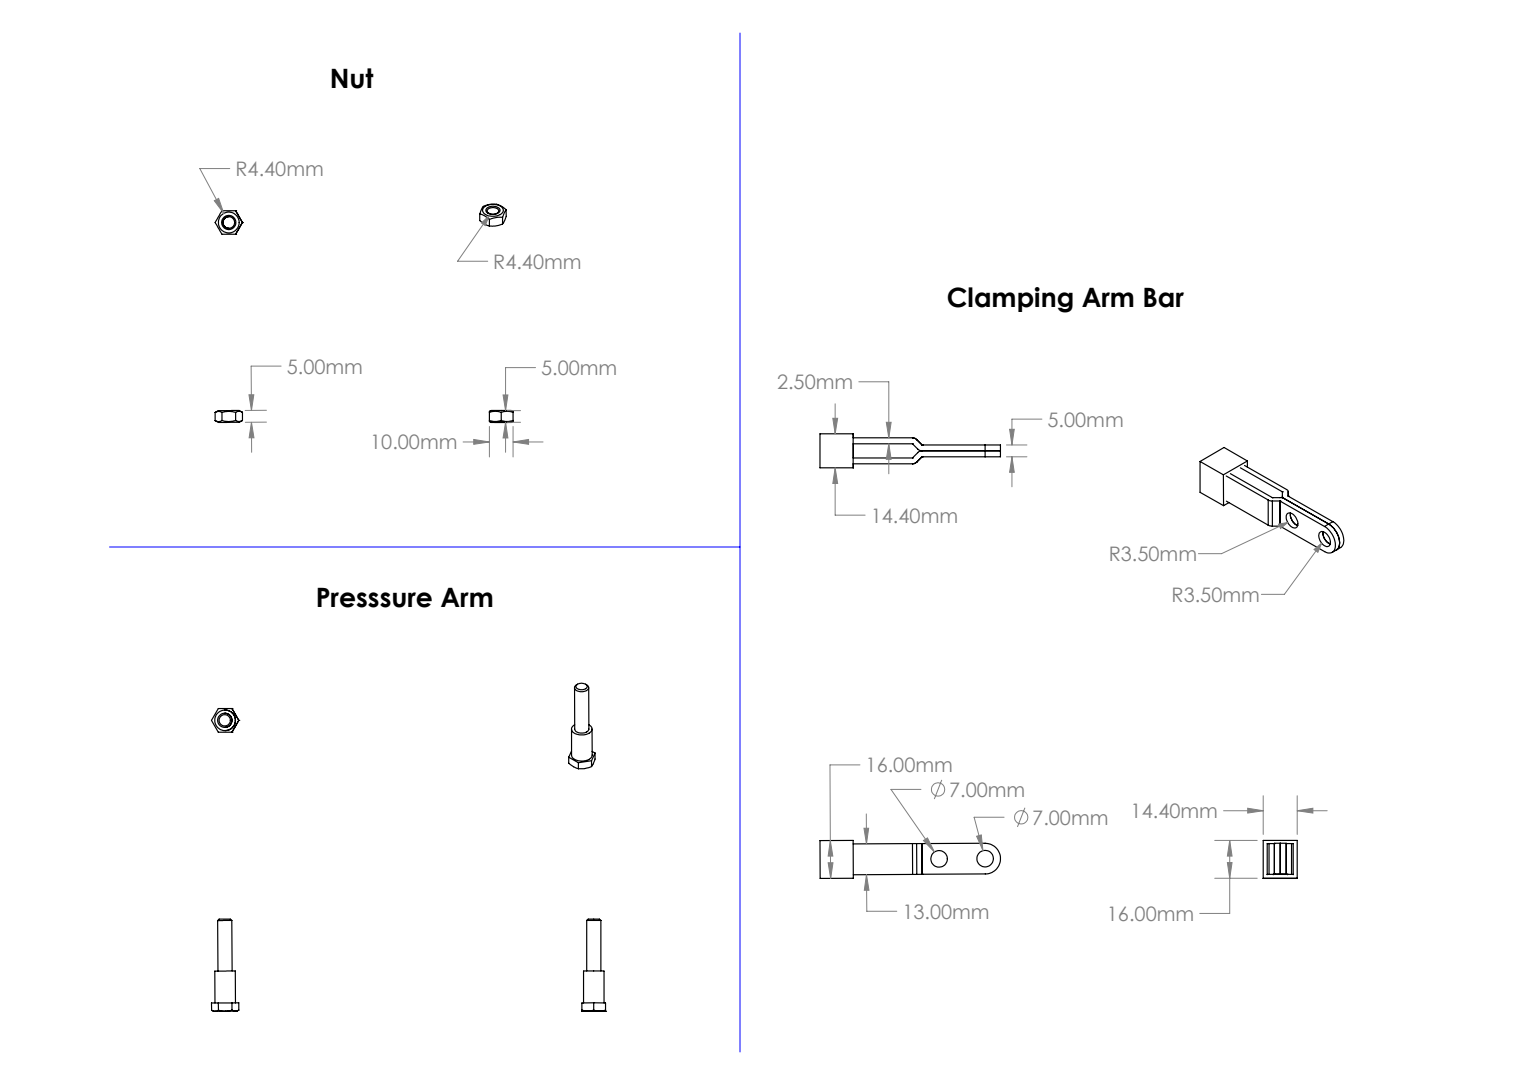
ISO-10303-21;
HEADER;
FILE_DESCRIPTION (('STEP AP203'),
    '1' );
FILE_NAME ('Nut.step',
    '2026-10-31T14:11:27',
    ( '' ),
    ( '' ),
    'SwSTEP 2.0',
    'SolidWorks 2024',
    '' );
FILE_SCHEMA (( 'AUTOMOTIVE_DESIGN' ));
ENDSEC;

DATA;
#48=ORIENTED_EDGE ( 'NONE', *, *, #17410, .F. ) ;
#83=EDGE_CURVE ( 'NONE', #7095, #13655, #23162, .T. ) ;
#118=EDGE_CURVE ( 'NONE', #1889, #6893, #1553, .T. ) ;
#162=CARTESIAN_POINT ( 'NONE',  ( -62.91331795724000386, 7.826945432762889787, -2.729132938682638176 ) ) ;
#166=DIRECTION ( 'NONE',  ( -0.005235963827117092427, 0.9999862922474493931, 2.636227439667000721E-16 ) ) ;
#193=ADVANCED_FACE ( 'NONE', ( #7501 ), #14386, .T. ) ;
#202=VECTOR ( 'NONE', #1831, 1000.000000000000114 ) ;
#242=ORIENTED_EDGE ( 'NONE', *, *, #2441, .T. ) ;
#415=DIRECTION ( 'NONE',  ( 1.000000000000000000, 0.000000000000000000, 0.000000000000000000 ) ) ;
#502=CONICAL_SURFACE ( 'NONE', #13794, 5.086751345948125724, 1.047197551196598297 ) ;
#564=ORIENTED_EDGE ( 'NONE', *, *, #13143, .F. ) ;
#585=ORIENTED_EDGE ( 'NONE', *, *, #14857, .F. ) ;
#607=DIRECTION ( 'NONE',  ( 0.002617981913558544045, -0.4999931461237241970, 0.8660254037844389297 ) ) ;
#658=ORIENTED_EDGE ( 'NONE', *, *, #17806, .F. ) ;
#748=FACE_OUTER_BOUND ( 'NONE', #10952, .T. ) ;
#759=FACE_OUTER_BOUND ( 'NONE', #8921, .T. ) ;
#769=CIRCLE ( 'NONE', #12189, 2.999765877365279998 ) ;
#838=ORIENTED_EDGE ( 'NONE', *, *, #7929, .T. ) ;
#909=( BOUNDED_CURVE ( )  B_SPLINE_CURVE ( 2, ( #15250, #2658, #18475 ),
 .UNSPECIFIED., .F., .F. ) 
 B_SPLINE_CURVE_WITH_KNOTS ( ( 3, 3 ),
 ( 0.000000000000000000, 0.5842180690389598974 ),
 .UNSPECIFIED. ) 
 CURVE ( )  GEOMETRIC_REPRESENTATION_ITEM ( )  RATIONAL_B_SPLINE_CURVE ( ( 1.000000000000000000, 1.154700538379259900, 1.000000000000000000 ) ) 
 REPRESENTATION_ITEM ( '' )  );
#924=APPLICATION_CONTEXT ( 'configuration controlled 3d designs of mechanical parts and assemblies' ) ;
#950=EDGE_CURVE ( 'NONE', #15424, #21777, #11621, .T. ) ;
#1004=DIRECTION ( 'NONE',  ( 0.000000000000000000, 0.000000000000000000, -1.000000000000000000 ) ) ;
#1008=VERTEX_POINT ( 'NONE', #8728 ) ;
#1066=ORIENTED_EDGE ( 'NONE', *, *, #2450, .T. ) ;
#1074=MECHANICAL_CONTEXT ( 'NONE', #3800, 'mechanical' ) ;
#1122=VECTOR ( 'NONE', #13490, 1000.000000000000114 ) ;
#1158=ORIENTED_EDGE ( 'NONE', *, *, #13143, .T. ) ;
#1192=ORIENTED_EDGE ( 'NONE', *, *, #14770, .T. ) ;
#1220=CARTESIAN_POINT ( 'NONE',  ( -62.91249983789198552, 7.670697574599230073, 2.108981951733699973E-15 ) ) ;
#1228=DIRECTION ( 'NONE',  ( 0.005235963827117092427, -0.9999862922474493931, -2.636227439667000721E-16 ) ) ;
#1258=( BOUNDED_CURVE ( )  B_SPLINE_CURVE ( 2, ( #13455, #15223, #2276 ),
 .UNSPECIFIED., .F., .F. ) 
 B_SPLINE_CURVE_WITH_KNOTS ( ( 3, 3 ),
 ( 0.000000000000000000, 0.5842180690389568998 ),
 .UNSPECIFIED. ) 
 CURVE ( )  GEOMETRIC_REPRESENTATION_ITEM ( )  RATIONAL_B_SPLINE_CURVE ( ( 1.000000000000000000, 1.154700538379249908, 1.000000000000000000 ) ) 
 REPRESENTATION_ITEM ( '' )  );
#1289=EDGE_LOOP ( 'NONE', ( #838, #3310, #5505, #18636 ) ) ;
#1334=CARTESIAN_POINT ( 'NONE',  ( -65.82539143210260590, 12.65551411021120032, 5.000000000000000000 ) ) ;
#1422=DIRECTION ( 'NONE',  ( 0.005235963827117092427, -0.9999862922474493931, -2.636227439667000721E-16 ) ) ;
#1439=CARTESIAN_POINT ( 'NONE',  ( -62.99678855639989905, 23.76850991288289805, -2.458499999999993690 ) ) ;
#1553=LINE ( 'NONE', #17616, #5745 ) ;
#1701=EDGE_LOOP ( 'NONE', ( #19939, #14934, #11313, #2927 ) ) ;
#1743=CARTESIAN_POINT ( 'NONE',  ( -62.93704341833160498, 12.35813331950920002, 2.458500000000117147 ) ) ;
#1749=DIRECTION ( 'NONE',  ( 0.9999862922474493931, 0.005235963827117055998, -1.750845403988397166E-31 ) ) ;
#1818=ORIENTED_EDGE ( 'NONE', *, *, #13921, .T. ) ;
#1831=DIRECTION ( 'NONE',  ( 0.002617981913558435191, -0.4999931461237237529, -0.8660254037844391517 ) ) ;
#1866=DIRECTION ( 'NONE',  ( 0.000000000000000000, 0.000000000000000000, -1.000000000000000000 ) ) ;
#1873=CARTESIAN_POINT ( 'NONE',  ( -57.16525610687759951, 12.70085888708699962, 5.715859474400029324E-15 ) ) ;
#1889=VERTEX_POINT ( 'NONE', #4406 ) ;
#1933=MANIFOLD_SOLID_BREP ( 'Imported1', #14367 ) ;
#2181=DIRECTION ( 'NONE',  ( -2.065223582182029992E-34, 2.636263576915770120E-16, -1.000000000000000000 ) ) ;
#2264=( GEOMETRIC_REPRESENTATION_CONTEXT ( 3 ) GLOBAL_UNCERTAINTY_ASSIGNED_CONTEXT ( ( #7928 ) ) GLOBAL_UNIT_ASSIGNED_CONTEXT ( ( #4646, #11789, #6547 ) ) REPRESENTATION_CONTEXT ( 'NONE', 'WORKASPACE' ) );
#2276=CARTESIAN_POINT ( 'NONE',  ( -60.04781580374580585, 11.89276268270289982, -5.000000000000000000 ) ) ;
#2301=DIRECTION ( 'NONE',  ( 0.005235963827117091560, -0.9999862922474493931, -2.636227439666999735E-16 ) ) ;
#2397=CIRCLE ( 'NONE', #19868, 4.399999999999997691 ) ;
#2419=ORIENTED_EDGE ( 'NONE', *, *, #15064, .T. ) ;
#2441=EDGE_CURVE ( 'NONE', #13655, #6050, #20011, .T. ) ;
#2450=EDGE_CURVE ( 'NONE', #13217, #14219, #21981, .T. ) ;
#2491=CARTESIAN_POINT ( 'NONE',  ( -57.16525610687759951, 12.70085888708699962, 5.715859474400029324E-15 ) ) ;
#2514=CARTESIAN_POINT ( 'NONE',  ( -65.82539143210260590, 12.65551411021120032, 5.000000000000000000 ) ) ;
#2569=CARTESIAN_POINT ( 'NONE',  ( 0.000000000000000000, 0.000000000000000000, 0.000000000000000000 ) ) ;
#2587=( BOUNDED_CURVE ( )  B_SPLINE_CURVE ( 2, ( #19385, #13684, #8344 ),
 .UNSPECIFIED., .F., .T. ) 
 B_SPLINE_CURVE_WITH_KNOTS ( ( 3, 3 ),
 ( 0.000000000000000000, 0.5842180690389588982 ),
 .UNSPECIFIED. ) 
 CURVE ( )  GEOMETRIC_REPRESENTATION_ITEM ( )  RATIONAL_B_SPLINE_CURVE ( ( 1.000000000000000000, 1.154700538379249908, 1.000000000000000000 ) ) 
 REPRESENTATION_ITEM ( '' )  );
#2605=EDGE_CURVE ( 'NONE', #22018, #17928, #909, .T. ) ;
#2653=AXIS2_PLACEMENT_3D ( 'NONE', #22839, #8363, #3007 ) ;
#2658=CARTESIAN_POINT ( 'NONE',  ( -67.24235627552212691, 7.607684554713951997, -2.500000000000000000 ) ) ;
#2677=CARTESIAN_POINT ( 'NONE',  ( -67.33861934291638818, 12.64759079499718375, 3.945395128240059864E-15 ) ) ;
#2734=ORIENTED_EDGE ( 'NONE', *, *, #4247, .F. ) ;
#2762=CARTESIAN_POINT ( 'NONE',  ( -62.99678855639989905, 23.76850991288289805, 2.458500000000006569 ) ) ;
#2799=ORIENTED_EDGE ( 'NONE', *, *, #10035, .T. ) ;
#2808=AXIS2_PLACEMENT_3D ( 'NONE', #14494, #21733, #5472 ) ;
#2809=ADVANCED_FACE ( 'NONE', ( #6343 ), #10163, .T. ) ;
#2822=EDGE_CURVE ( 'NONE', #1008, #6050, #7463, .T. ) ;
#2848=CARTESIAN_POINT ( 'NONE',  ( -60.04781580374580585, 11.89276268270289982, 5.000000000000000000 ) ) ;
#2856=ADVANCED_BREP_SHAPE_REPRESENTATION ( '', ( #1933, #12739 ), #2264 ) ;
#2927=ORIENTED_EDGE ( 'NONE', *, *, #18076, .T. ) ;
#2955=CARTESIAN_POINT ( 'NONE',  ( -60.04781580374580585, 11.89276268270289982, 5.000000000000000000 ) ) ;
#2961=DIRECTION ( 'NONE',  ( -0.005235963827117092427, 0.9999862922474493931, 2.636227439667000721E-16 ) ) ;
#3007=DIRECTION ( 'NONE',  ( 0.9999862922474493931, 0.005235963827117055998, -1.750845403988397166E-31 ) ) ;
#3099=ORIENTED_EDGE ( 'NONE', *, *, #10881, .F. ) ;
#3193=EDGE_CURVE ( 'NONE', #17928, #13217, #16240, .T. ) ;
#3195=CARTESIAN_POINT ( 'NONE',  ( -68.69007546624879978, 8.433449002107520798, 2.873144230283079984E-15 ) ) ;
#3310=ORIENTED_EDGE ( 'NONE', *, *, #950, .T. ) ;
#3325=FACE_OUTER_BOUND ( 'NONE', #4037, .T. ) ;
#3450=CARTESIAN_POINT ( 'NONE',  ( -62.99678855639989905, 23.76850991288289805, 6.352789585277969841E-15 ) ) ;
#3602=CARTESIAN_POINT ( 'NONE',  ( -67.26895854462254931, 12.68829727884599201, -2.499999999999999556 ) ) ;
#3687=AXIS2_PLACEMENT_3D ( 'NONE', #13492, #20727, #5393 ) ;
#3754=DIRECTION ( 'NONE',  ( 0.9999862922474491711, 0.005235963827117207786, -1.514467536079854800E-31 ) ) ;
#3762=ORIENTED_EDGE ( 'NONE', *, *, #4612, .F. ) ;
#3800=APPLICATION_CONTEXT ( 'configuration controlled 3d designs of mechanical parts and assemblies' ) ;
#3801=DIRECTION ( 'NONE',  ( 0.005235963827117092427, -0.9999862922474493931, -2.636227439667000721E-16 ) ) ;
#3816=ADVANCED_FACE ( 'NONE', ( #5637 ), #12564, .F. ) ;
#3882=AXIS2_PLACEMENT_3D ( 'NONE', #15257, #11723, #9577 ) ;
#4033=DIRECTION ( 'NONE',  ( 0.005235963827117092427, -0.9999862922474493931, -2.636227439667000721E-16 ) ) ;
#4037=EDGE_LOOP ( 'NONE', ( #2734, #6715, #5931, #12250 ) ) ;
#4108=CARTESIAN_POINT ( 'NONE',  ( -65.80336369117380002, 8.448563927732790191, -5.000000000000000000 ) ) ;
#4131=FACE_OUTER_BOUND ( 'NONE', #11927, .T. ) ;
#4152=CARTESIAN_POINT ( 'NONE',  ( -58.58222095029707077, 7.653029331589754847, 2.499999999999999556 ) ) ;
#4184=CARTESIAN_POINT ( 'NONE',  ( -68.71210320717760567, 12.64039918458589895, 4.433884350144319916E-15 ) ) ;
#4247=EDGE_CURVE ( 'NONE', #15424, #7095, #16030, .T. ) ;
#4308=ORIENTED_EDGE ( 'NONE', *, *, #10796, .T. ) ;
#4336=FACE_OUTER_BOUND ( 'NONE', #12032, .T. ) ;
#4406=CARTESIAN_POINT ( 'NONE',  ( -58.51256015200321059, 7.693735815438545345, 2.108981951733699184E-15 ) ) ;
#4413=LINE ( 'NONE', #2514, #14045 ) ;
#4482=EDGE_CURVE ( 'NONE', #15538, #1008, #9896, .T. ) ;
#4520=CARTESIAN_POINT ( 'NONE',  ( -60.04781580374580585, 11.89276268270289982, -5.000000000000000000 ) ) ;
#4546=AXIS2_PLACEMENT_3D ( 'NONE', #13889, #2961, #6776 ) ;
#4568=ADVANCED_FACE ( 'NONE', ( #22220 ), #5965, .T. ) ;
#4593=( BOUNDED_CURVE ( )  B_SPLINE_CURVE ( 2, ( #9269, #9752, #20191 ),
 .UNSPECIFIED., .F., .F. ) 
 B_SPLINE_CURVE_WITH_KNOTS ( ( 3, 3 ),
 ( 0.000000000000000000, 0.5842180690389568998 ),
 .UNSPECIFIED. ) 
 CURVE ( )  GEOMETRIC_REPRESENTATION_ITEM ( )  RATIONAL_B_SPLINE_CURVE ( ( 1.000000000000000000, 1.154700538379249908, 1.000000000000000000 ) ) 
 REPRESENTATION_ITEM ( '' )  );
#4612=EDGE_CURVE ( 'NONE', #15424, #15538, #15813, .T. ) ;
#4618=VECTOR ( 'NONE', #15931, 1000.000000000000000 ) ;
#4630=DIRECTION ( 'NONE',  ( -0.002617981913558544045, 0.4999931461237241970, -0.8660254037844389297 ) ) ;
#4646=( LENGTH_UNIT ( ) NAMED_UNIT ( * ) SI_UNIT ( .MILLI., .METRE. ) );
#4714=ORIENTED_EDGE ( 'NONE', *, *, #3193, .F. ) ;
#4771=LINE ( 'NONE', #16801, #18748 ) ;
#4897=CARTESIAN_POINT ( 'NONE',  ( -65.82123935389580538, 11.86253283145240012, 5.000000000000000000 ) ) ;
#5071=CARTESIAN_POINT ( 'NONE',  ( -62.91413607658799378, 7.983193290926558383, 2.191364059223300011E-15 ) ) ;
#5115=CARTESIAN_POINT ( 'NONE',  ( -62.99678855639989905, 23.76850991288289805, 6.352789585277969841E-15 ) ) ;
#5160=EDGE_CURVE ( 'NONE', #21777, #22844, #7220, .T. ) ;
#5174=DIRECTION ( 'NONE',  ( 0.000000000000000000, 0.000000000000000000, 1.000000000000000000 ) ) ;
#5204=CARTESIAN_POINT ( 'NONE',  ( -67.24235627552209849, 7.607684554713948444, 2.499999999999999556 ) ) ;
#5240=EDGE_CURVE ( 'NONE', #7095, #22844, #15320, .T. ) ;
#5281=CARTESIAN_POINT ( 'NONE',  ( -60.02994014102380049, 8.478793778983318319, -5.000000000000000000 ) ) ;
#5326=CARTESIAN_POINT ( 'NONE',  ( -57.14322836594880073, 8.493908704608589488, 2.318032717970499742E-15 ) ) ;
#5393=DIRECTION ( 'NONE',  ( 6.009176021521548497E-19, -0.9999588795606765279, 0.009068582455730085992 ) ) ;
#5433=CARTESIAN_POINT ( 'NONE',  ( -62.93660361792420588, 12.27413839645710070, 3.322570288448809768E-15 ) ) ;
#5438=AXIS2_PLACEMENT_3D ( 'NONE', #9077, #23323, #11120 ) ;
#5472=DIRECTION ( 'NONE',  ( 0.000000000000000000, 0.000000000000000000, 1.000000000000000000 ) ) ;
#5505=ORIENTED_EDGE ( 'NONE', *, *, #5160, .T. ) ;
#5618=ORIENTED_EDGE ( 'NONE', *, *, #21166, .F. ) ;
#5637=FACE_OUTER_BOUND ( 'NONE', #1701, .T. ) ;
#5745=VECTOR ( 'NONE', #8823, 1000.000000000000114 ) ;
#5757=CARTESIAN_POINT ( 'NONE',  ( -62.93786153767959490, 12.51438117767279934, 3.385904617822409831E-15 ) ) ;
#5783=FACE_OUTER_BOUND ( 'NONE', #17641, .T. ) ;
#5803=AXIS2_PLACEMENT_3D ( 'NONE', #9495, #19949, #14953 ) ;
#5818=AXIS2_PLACEMENT_3D ( 'NONE', #5115, #23377, #14247 ) ;
#5931=ORIENTED_EDGE ( 'NONE', *, *, #10263, .F. ) ;
#5965=PLANE ( 'NONE',  #15646 ) ;
#5993=FACE_BOUND ( 'NONE', #23430, .T. ) ;
#6034=CARTESIAN_POINT ( 'NONE',  ( -62.93704341833160498, 12.35813331950920002, -2.458500000000113150 ) ) ;
#6050=VERTEX_POINT ( 'NONE', #11465 ) ;
#6159=AXIS2_PLACEMENT_3D ( 'NONE', #11289, #10611, #18518 ) ;
#6199=EDGE_CURVE ( 'NONE', #11763, #11453, #2587, .T. ) ;
#6237=CARTESIAN_POINT ( 'NONE',  ( -60.02994014102380049, 8.478793778983318319, -5.000000000000000000 ) ) ;
#6239=FACE_OUTER_BOUND ( 'NONE', #9069, .T. ) ;
#6250=PLANE ( 'NONE',  #3687 ) ;
#6252=EDGE_CURVE ( 'NONE', #11453, #23172, #19441, .T. ) ;
#6318=CARTESIAN_POINT ( 'NONE',  ( -62.91331795724000386, 7.826945432762889787, 2.729132938682642617 ) ) ;
#6337=FACE_OUTER_BOUND ( 'NONE', #9256, .T. ) ;
#6343=FACE_OUTER_BOUND ( 'NONE', #13109, .T. ) ;
#6400=ORIENTED_EDGE ( 'NONE', *, *, #21166, .T. ) ;
#6414=CARTESIAN_POINT ( 'NONE',  ( -62.91331795724000386, 7.826945432762889787, 2.150173005478499992E-15 ) ) ;
#6491=EDGE_LOOP ( 'NONE', ( #9619, #22336, #18153, #15288 ) ) ;
#6547=( NAMED_UNIT ( * ) SI_UNIT ( $, .STERADIAN. ) SOLID_ANGLE_UNIT ( ) );
#6715=ORIENTED_EDGE ( 'NONE', *, *, #4612, .T. ) ;
#6776=DIRECTION ( 'NONE',  ( 0.000000000000000000, 0.000000000000000000, -1.000000000000000000 ) ) ;
#6793=ADVANCED_FACE ( 'NONE', ( #11913 ), #21721, .F. ) ;
#6797=CYLINDRICAL_SURFACE ( 'NONE', #21711, 2.458500000000000352 ) ;
#6893=VERTEX_POINT ( 'NONE', #5326 ) ;
#6975=PLANE ( 'NONE',  #5438 ) ;
#7032=FACE_OUTER_BOUND ( 'NONE', #11934, .T. ) ;
#7034=CARTESIAN_POINT ( 'NONE',  ( -65.82123935389580538, 11.86253283145240012, 5.000000000000000000 ) ) ;
#7095=VERTEX_POINT ( 'NONE', #6034 ) ;
#7220=CIRCLE ( 'NONE', #4546, 2.999765877365279998 ) ;
#7238=ORIENTED_EDGE ( 'NONE', *, *, #6199, .T. ) ;
#7257=AXIS2_PLACEMENT_3D ( 'NONE', #9569, #22596, #15367 ) ;
#7338=CIRCLE ( 'NONE', #5803, 2.458500000000000352 ) ;
#7358=DIRECTION ( 'NONE',  ( -0.005235963827117092427, 0.9999862922474493931, 2.636227439667000721E-16 ) ) ;
#7375=CIRCLE ( 'NONE', #2808, 2.458500000000000352 ) ;
#7377=ADVANCED_FACE ( 'NONE', ( #21653 ), #6975, .T. ) ;
#7463=CIRCLE ( 'NONE', #10513, 2.999765877365279998 ) ;
#7501=FACE_OUTER_BOUND ( 'NONE', #13056, .T. ) ;
#7530=ORIENTED_EDGE ( 'NONE', *, *, #14770, .F. ) ;
#7547=CIRCLE ( 'NONE', #16254, 4.399999999999997691 ) ;
#7614=PRODUCT_DEFINITION_FORMATION_WITH_SPECIFIED_SOURCE ( 'ANY', '', #21422, .NOT_KNOWN. ) ;
#7711=ADVANCED_FACE ( 'NONE', ( #3325 ), #16031, .F. ) ;
#7842=ORIENTED_EDGE ( 'NONE', *, *, #16626, .T. ) ;
#7879=DIRECTION ( 'NONE',  ( -0.005235963827117002221, 0.9999862922474493931, 2.636227439667000721E-16 ) ) ;
#7928=UNCERTAINTY_MEASURE_WITH_UNIT (LENGTH_MEASURE( 1.000000000000000082E-05 ), #4646, 'distance_accuracy_value', 'NONE');
#7929=EDGE_CURVE ( 'NONE', #7095, #15424, #7338, .T. ) ;
#8023=PLANE ( 'NONE',  #3882 ) ;
#8278=CARTESIAN_POINT ( 'NONE',  ( -62.91413607658799378, 7.983193290926554830, -2.458499999999998131 ) ) ;
#8326=ORIENTED_EDGE ( 'NONE', *, *, #17806, .T. ) ;
#8344=CARTESIAN_POINT ( 'NONE',  ( -65.82123935389580538, 11.86253283145240012, 5.000000000000000000 ) ) ;
#8363=DIRECTION ( 'NONE',  ( 0.005235963827117002221, -0.9999862922474493931, -2.636227439667000721E-16 ) ) ;
#8394=AXIS2_PLACEMENT_3D ( 'NONE', #5071, #10437, #5174 ) ;
#8521=ADVANCED_FACE ( 'NONE', ( #5783 ), #502, .T. ) ;
#8551=CARTESIAN_POINT ( 'NONE',  ( -65.80336369117380002, 8.448563927732790191, 5.000000000000000000 ) ) ;
#8631=AXIS2_PLACEMENT_3D ( 'NONE', #1220, #15484, #22711 ) ;
#8686=DIRECTION ( 'NONE',  ( 0.000000000000000000, -2.891431443143872083E-16, 1.000000000000000000 ) ) ;
#8720=ORIENTED_EDGE ( 'NONE', *, *, #15064, .F. ) ;
#8728=CARTESIAN_POINT ( 'NONE',  ( -62.91249983789201394, 7.670697574599229185, 2.999765877365274225 ) ) ;
#8737=FACE_OUTER_BOUND ( 'NONE', #1289, .T. ) ;
#8820=AXIS2_PLACEMENT_3D ( 'NONE', #5757, #166, #19783 ) ;
#8823=DIRECTION ( 'NONE',  ( 0.8633955506089426857, 0.5045276238113038936, 1.318113719833497156E-16 ) ) ;
#8833=ADVANCED_FACE ( 'NONE', ( #8737 ), #11568, .F. ) ;
#8843=CARTESIAN_POINT ( 'NONE',  ( -62.91249983789198552, 7.670697574599230073, 2.108981951733699973E-15 ) ) ;
#8878=EDGE_LOOP ( 'NONE', ( #13461, #6400, #15152, #13059 ) ) ;
#8905=CARTESIAN_POINT ( 'NONE',  ( -62.93867965702761325, 12.67062903583649991, 3.427095671567209849E-15 ) ) ;
#8921=EDGE_LOOP ( 'NONE', ( #8326, #21308, #7842, #14062 ) ) ;
#8926=DIRECTION ( 'NONE',  ( 0.005235963827117092427, -0.9999862922474493931, -2.636227439667000721E-16 ) ) ;
#8927=ORIENTED_EDGE ( 'NONE', *, *, #14857, .T. ) ;
#9031=ORIENTED_EDGE ( 'NONE', *, *, #17769, .F. ) ;
#9040=ORIENTED_EDGE ( 'NONE', *, *, #118, .F. ) ;
#9069=EDGE_LOOP ( 'NONE', ( #21735, #4308 ) ) ;
#9077=CARTESIAN_POINT ( 'NONE',  ( -60.05196788195259927, 12.68574396146170180, -5.000000000000000000 ) ) ;
#9187=ORIENTED_EDGE ( 'NONE', *, *, #13271, .T. ) ;
#9256=EDGE_LOOP ( 'NONE', ( #15488, #18036, #20908, #19383, #14472, #4714 ) ) ;
#9269=CARTESIAN_POINT ( 'NONE',  ( -60.02994014102380049, 8.478793778983318319, -5.000000000000000000 ) ) ;
#9274=CARTESIAN_POINT ( 'NONE',  ( -67.31243952378076756, 7.647659333759914801, 1.570137360108866347E-15 ) ) ;
#9346=CARTESIAN_POINT ( 'NONE',  ( -62.93867965702761325, 12.67062903583649991, 3.427095671567209849E-15 ) ) ;
#9495=CARTESIAN_POINT ( 'NONE',  ( -62.93704341833160498, 12.35813331950920002, 3.344713564077609812E-15 ) ) ;
#9536=ORIENTED_EDGE ( 'NONE', *, *, #6199, .F. ) ;
#9558=EDGE_CURVE ( 'NONE', #11453, #13217, #4413, .T. ) ;
#9569=CARTESIAN_POINT ( 'NONE',  ( -62.91249983789198552, 7.670697574599230073, 2.731378056153440284E-17 ) ) ;
#9577=DIRECTION ( 'NONE',  ( -0.5000051404512477760, 0.000000000000000000, 0.8660224359231856184 ) ) ;
#9619=ORIENTED_EDGE ( 'NONE', *, *, #2441, .F. ) ;
#9752=CARTESIAN_POINT ( 'NONE',  ( -62.91228861290962726, 7.630356943151859639, -4.999999999999999112 ) ) ;
#9896=LINE ( 'NONE', #6318, #20941 ) ;
#10011=DIRECTION ( 'NONE',  ( 0.000000000000000000, 0.000000000000000000, 1.000000000000000000 ) ) ;
#10035=EDGE_CURVE ( 'NONE', #6050, #1008, #769, .T. ) ;
#10131=DIRECTION ( 'NONE',  ( 0.005235963827117092427, -0.9999862922474493931, -2.636227439667000721E-16 ) ) ;
#10163=PLANE ( 'NONE',  #20730 ) ;
#10263=EDGE_CURVE ( 'NONE', #13655, #15538, #11015, .T. ) ;
#10311=ORIENTED_EDGE ( 'NONE', *, *, #83, .T. ) ;
#10346=CARTESIAN_POINT ( 'NONE',  ( -62.93786153767959490, 12.51438117767279934, -2.729132938682636844 ) ) ;
#10350=ORIENTED_EDGE ( 'NONE', *, *, #18076, .F. ) ;
#10405=DIRECTION ( 'NONE',  ( -3.638785342205658653E-34, -2.636191302913590118E-16, 1.000000000000000000 ) ) ;
#10437=DIRECTION ( 'NONE',  ( -0.005235963827117092427, 0.9999862922474493931, 2.636227439667000721E-16 ) ) ;
#10513=AXIS2_PLACEMENT_3D ( 'NONE', #8843, #11093, #12748 ) ;
#10522=VERTEX_POINT ( 'NONE', #5281 ) ;
#10545=ORIENTED_EDGE ( 'NONE', *, *, #10796, .F. ) ;
#10611=DIRECTION ( 'NONE',  ( 0.005235963827117092427, -0.9999862922474493931, -2.636227439667000721E-16 ) ) ;
#10613=ADVANCED_FACE ( 'NONE', ( #6239, #5993 ), #11718, .T. ) ;
#10796=EDGE_CURVE ( 'NONE', #16722, #1889, #11784, .T. ) ;
#10809=CARTESIAN_POINT ( 'NONE',  ( -62.91413607658799378, 7.983193290926554830, 2.458500000000002572 ) ) ;
#10817=ORIENTED_EDGE ( 'NONE', *, *, #19963, .T. ) ;
#10864=EDGE_CURVE ( 'NONE', #1889, #16722, #23024, .T. ) ;
#10881=EDGE_CURVE ( 'NONE', #23172, #13198, #17778, .T. ) ;
#10952=EDGE_LOOP ( 'NONE', ( #11285, #8927, #12887, #5618 ) ) ;
#11012=VERTEX_POINT ( 'NONE', #14527 ) ;
#11015=CIRCLE ( 'NONE', #8394, 2.458500000000000352 ) ;
#11025=VECTOR ( 'NONE', #4630, 1000.000000000000114 ) ;
#11093=DIRECTION ( 'NONE',  ( 0.005235963827117092427, -0.9999862922474493931, -2.636227439667000721E-16 ) ) ;
#11097=VERTEX_POINT ( 'NONE', #22570 ) ;
#11120=DIRECTION ( 'NONE',  ( -9.096131349985791167E-47, -1.000000000000000000, -2.757014059715200372E-16 ) ) ;
#11285=ORIENTED_EDGE ( 'NONE', *, *, #10881, .T. ) ;
#11289=CARTESIAN_POINT ( 'NONE',  ( -62.93660361792420588, 12.27413839645710070, 3.322570288448809768E-15 ) ) ;
#11313=ORIENTED_EDGE ( 'NONE', *, *, #5240, .T. ) ;
#11423=CARTESIAN_POINT ( 'NONE',  ( -57.14322836594880073, 8.493908704608589488, 2.318032717970499742E-15 ) ) ;
#11453=VERTEX_POINT ( 'NONE', #7034 ) ;
#11459=DIRECTION ( 'NONE',  ( -0.8660135325225010172, -0.004534477687579933393, 0.5000000000000001110 ) ) ;
#11465=CARTESIAN_POINT ( 'NONE',  ( -62.91249983789201394, 7.670697574599230961, -2.999765877365268008 ) ) ;
#11519=EDGE_LOOP ( 'NONE', ( #10350, #14839 ) ) ;
#11568=CONICAL_SURFACE ( 'NONE', #22899, 2.729132938682640397, 1.047197551196598297 ) ;
#11603=PLANE ( 'NONE',  #21908 ) ;
#11621=LINE ( 'NONE', #15378, #1122 ) ;
#11631=EDGE_CURVE ( 'NONE', #11097, #6893, #16607, .T. ) ;
#11684=CARTESIAN_POINT ( 'NONE',  ( -60.05196788195259927, 12.68574396146170180, -5.000000000000000000 ) ) ;
#11691=AXIS2_PLACEMENT_3D ( 'NONE', #21601, #12487, #14143 ) ;
#11702=DIRECTION ( 'NONE',  ( 0.9999862922474491711, 0.005235963827116866913, -1.514467536079854800E-31 ) ) ;
#11714=CARTESIAN_POINT ( 'NONE',  ( -57.14322836594880073, 8.493908704608589488, 2.318032717970499742E-15 ) ) ;
#11718=PLANE ( 'NONE',  #7257 ) ;
#11723=DIRECTION ( 'NONE',  ( -0.8660135325225002401, -0.004534477687579664511, -0.5000000000000014433 ) ) ;
#11751=LINE ( 'NONE', #13750, #14866 ) ;
#11763=VERTEX_POINT ( 'NONE', #2955 ) ;
#11784=CIRCLE ( 'NONE', #2653, 4.399999999999997691 ) ;
#11789=( NAMED_UNIT ( * ) PLANE_ANGLE_UNIT ( ) SI_UNIT ( $, .RADIAN. ) );
#11792=CARTESIAN_POINT ( 'NONE',  ( -65.82123935389580538, 11.86253283145240012, -5.000000000000000000 ) ) ;
#11913=FACE_OUTER_BOUND ( 'NONE', #6491, .T. ) ;
#11927=EDGE_LOOP ( 'NONE', ( #48, #18297, #10817, #564, #16772, #3099 ) ) ;
#11934=EDGE_LOOP ( 'NONE', ( #15975, #242, #2799, #18790 ) ) ;
#12027=CARTESIAN_POINT ( 'NONE',  ( -57.16110402867079898, 11.90787760832819941, 3.218044905330409686E-15 ) ) ;
#12032=EDGE_LOOP ( 'NONE', ( #9187, #15734 ) ) ;
#12036=DIRECTION ( 'NONE',  ( -0.8633955506089426857, -0.5045276238113038936, -2.575384811085907648E-17 ) ) ;
#12079=ORIENTED_EDGE ( 'NONE', *, *, #2605, .F. ) ;
#12189=AXIS2_PLACEMENT_3D ( 'NONE', #20282, #1422, #8686 ) ;
#12250=ORIENTED_EDGE ( 'NONE', *, *, #83, .F. ) ;
#12255=VECTOR ( 'NONE', #1228, 1000.000000000000000 ) ;
#12329=CARTESIAN_POINT ( 'NONE',  ( -62.93786153767959490, 12.51438117767279934, 3.385904617822409831E-15 ) ) ;
#12439=CONICAL_SURFACE ( 'NONE', #11691, 2.729132938682640397, 1.047197551196598297 ) ;
#12444=ADVANCED_FACE ( 'NONE', ( #4336, #18468 ), #11603, .F. ) ;
#12465=CARTESIAN_POINT ( 'NONE',  ( -68.69007546624879978, 8.433449002107520798, 2.873144230283079984E-15 ) ) ;
#12487=DIRECTION ( 'NONE',  ( 0.005235963827117092427, -0.9999862922474493931, -2.636227439667000721E-16 ) ) ;
#12564=CONICAL_SURFACE ( 'NONE', #8820, 2.729132938682640397, 1.047197551196598297 ) ;
#12628=VECTOR ( 'NONE', #15704, 1000.000000000000000 ) ;
#12642=ADVANCED_FACE ( 'NONE', ( #6337 ), #16996, .T. ) ;
#12725=DIRECTION ( 'NONE',  ( 0.000000000000000000, 0.000000000000000000, -1.000000000000000000 ) ) ;
#12739=AXIS2_PLACEMENT_3D ( 'NONE', #2569, #13380, #415 ) ;
#12748=DIRECTION ( 'NONE',  ( 0.000000000000000000, -2.891431443143872083E-16, 1.000000000000000000 ) ) ;
#12881=CARTESIAN_POINT ( 'NONE',  ( -62.91228861290962726, 7.630356943151853422, 4.999999999999999112 ) ) ;
#12887=ORIENTED_EDGE ( 'NONE', *, *, #2605, .T. ) ;
#12912=CARTESIAN_POINT ( 'NONE',  ( -68.00125749501478367, 8.040554167933716911, 1.590559959464714451E-15 ) ) ;
#13040=DIRECTION ( 'NONE',  ( 0.005235963827117092427, -0.9999862922474493931, -2.636227439667000721E-16 ) ) ;
#13056=EDGE_LOOP ( 'NONE', ( #1158, #21020, #1818, #7530 ) ) ;
#13059=ORIENTED_EDGE ( 'NONE', *, *, #9558, .F. ) ;
#13109=EDGE_LOOP ( 'NONE', ( #7238, #17714, #1066, #14357 ) ) ;
#13143=EDGE_CURVE ( 'NONE', #20578, #11097, #20961, .T. ) ;
#13188=CARTESIAN_POINT ( 'NONE',  ( -60.02994014102380049, 8.478793778983318319, 5.000000000000000000 ) ) ;
#13198=VERTEX_POINT ( 'NONE', #11792 ) ;
#13217=VERTEX_POINT ( 'NONE', #20790 ) ;
#13271=EDGE_CURVE ( 'NONE', #11012, #22086, #7547, .T. ) ;
#13339=ORIENTED_EDGE ( 'NONE', *, *, #17029, .F. ) ;
#13380=DIRECTION ( 'NONE',  ( 0.000000000000000000, 0.000000000000000000, 1.000000000000000000 ) ) ;
#13455=CARTESIAN_POINT ( 'NONE',  ( -65.82123935389580538, 11.86253283145240012, -5.000000000000000000 ) ) ;
#13461=ORIENTED_EDGE ( 'NONE', *, *, #6252, .T. ) ;
#13490=DIRECTION ( 'NONE',  ( -0.002617981913558647261, 0.4999931461237237529, 0.8660254037844391517 ) ) ;
#13492=CARTESIAN_POINT ( 'NONE',  ( -60.05196788195259927, 12.68574396146170180, 5.000000000000000000 ) ) ;
#13655=VERTEX_POINT ( 'NONE', #8278 ) ;
#13684=CARTESIAN_POINT ( 'NONE',  ( -62.93889088200999282, 12.71096966728388722, 4.999999999999999112 ) ) ;
#13732=DIRECTION ( 'NONE',  ( -0.005235963827117092427, 0.9999862922474493931, 2.636227439667000721E-16 ) ) ;
#13750=CARTESIAN_POINT ( 'NONE',  ( -57.84992199990481510, 12.30077244250202462, 3.322570288448809374E-15 ) ) ;
#13794=AXIS2_PLACEMENT_3D ( 'NONE', #5433, #13040, #3754 ) ;
#13834=DIRECTION ( 'NONE',  ( 0.005235963827117092427, -0.9999862922474493931, -2.636227439667000721E-16 ) ) ;
#13889=CARTESIAN_POINT ( 'NONE',  ( -62.93867965702761325, 12.67062903583649991, 3.427095671567209849E-15 ) ) ;
#13908=LINE ( 'NONE', #22681, #16203 ) ;
#13921=EDGE_CURVE ( 'NONE', #6893, #10522, #16376, .T. ) ;
#14017=PRODUCT_DEFINITION_SHAPE ( 'NONE', 'NONE',  #22291 ) ;
#14043=CARTESIAN_POINT ( 'NONE',  ( -62.93867965702758482, 12.67062903583650169, -2.999765877365338174 ) ) ;
#14045=VECTOR ( 'NONE', #16755, 1000.000000000000000 ) ;
#14062=ORIENTED_EDGE ( 'NONE', *, *, #11631, .F. ) ;
#14114=EDGE_LOOP ( 'NONE', ( #10545, #19802, #12079, #8720, #18919, #9040 ) ) ;
#14143=DIRECTION ( 'NONE',  ( 0.000000000000000000, 0.000000000000000000, 1.000000000000000000 ) ) ;
#14219=VERTEX_POINT ( 'NONE', #19401 ) ;
#14247=DIRECTION ( 'NONE',  ( 0.000000000000000000, 0.000000000000000000, -1.000000000000000000 ) ) ;
#14357=ORIENTED_EDGE ( 'NONE', *, *, #19019, .F. ) ;
#14367=CLOSED_SHELL ( 'NONE', ( #20826, #8521, #14939, #7711, #8833, #3816, #16375, #12444, #6793, #10613, #19784, #12642, #193, #7377, #22222, #2809, #18864, #4568 ) ) ;
#14386=PLANE ( 'NONE',  #19913 ) ;
#14472=ORIENTED_EDGE ( 'NONE', *, *, #2450, .F. ) ;
#14494=CARTESIAN_POINT ( 'NONE',  ( -62.91413607658799378, 7.983193290926558383, 2.191364059223300011E-15 ) ) ;
#14516=AXIS2_PLACEMENT_3D ( 'NONE', #6414, #19143, #10011 ) ;
#14527=CARTESIAN_POINT ( 'NONE',  ( -58.53873997113881700, 12.69366727667581429, 3.427095671567204722E-15 ) ) ;
#14770=EDGE_CURVE ( 'NONE', #20578, #10522, #15566, .T. ) ;
#14776=CARTESIAN_POINT ( 'NONE',  ( -58.58222095029707077, 7.653029331589754847, -2.499999999999991118 ) ) ;
#14804=DIRECTION ( 'NONE',  ( -0.005235963827117092427, 0.9999862922474493931, 2.636227439667000721E-16 ) ) ;
#14839=ORIENTED_EDGE ( 'NONE', *, *, #5160, .F. ) ;
#14857=EDGE_CURVE ( 'NONE', #13198, #22018, #13908, .T. ) ;
#14866=VECTOR ( 'NONE', #17203, 1000.000000000000114 ) ;
#14934=ORIENTED_EDGE ( 'NONE', *, *, #4247, .T. ) ;
#14939=ADVANCED_FACE ( 'NONE', ( #7032 ), #12439, .F. ) ;
#14953=DIRECTION ( 'NONE',  ( 0.000000000000000000, 0.000000000000000000, -1.000000000000000000 ) ) ;
#15064=EDGE_CURVE ( 'NONE', #10522, #22018, #4593, .T. ) ;
#15106=DIRECTION ( 'NONE',  ( -0.005235963827117252022, 0.9999862922474493931, 3.469446951953616307E-19 ) ) ;
#15114=CARTESIAN_POINT ( 'NONE',  ( -62.91457587699539289, 8.067188213978639055, 2.213507334852100055E-15 ) ) ;
#15152=ORIENTED_EDGE ( 'NONE', *, *, #3193, .T. ) ;
#15223=CARTESIAN_POINT ( 'NONE',  ( -62.93889088200999282, 12.71096966728388722, -4.999999999999999112 ) ) ;
#15250=CARTESIAN_POINT ( 'NONE',  ( -65.80336369117380002, 8.448563927732790191, -5.000000000000000000 ) ) ;
#15257=CARTESIAN_POINT ( 'NONE',  ( -65.82539143210260590, 12.65551411021120032, -5.000000000000000000 ) ) ;
#15288=ORIENTED_EDGE ( 'NONE', *, *, #2822, .T. ) ;
#15320=LINE ( 'NONE', #10346, #11025 ) ;
#15335=CARTESIAN_POINT ( 'NONE',  ( -58.60882321939752160, 12.73364205572179841, -2.499999999999991118 ) ) ;
#15353=FACE_OUTER_BOUND ( 'NONE', #14114, .T. ) ;
#15361=DIRECTION ( 'NONE',  ( 0.9999862922474491711, 0.005235963827116866913, -1.514467536079854800E-31 ) ) ;
#15367=DIRECTION ( 'NONE',  ( -2.065223582182029992E-34, 2.636263576915770120E-16, -1.000000000000000000 ) ) ;
#15378=CARTESIAN_POINT ( 'NONE',  ( -62.93786153767959490, 12.51438117767279934, 2.729132938682643950 ) ) ;
#15424=VERTEX_POINT ( 'NONE', #1743 ) ;
#15484=DIRECTION ( 'NONE',  ( 0.005235963827117002221, -0.9999862922474493931, -2.636227439667000721E-16 ) ) ;
#15488=ORIENTED_EDGE ( 'NONE', *, *, #21592, .F. ) ;
#15538=VERTEX_POINT ( 'NONE', #10809 ) ;
#15566=LINE ( 'NONE', #11684, #16575 ) ;
#15593=CARTESIAN_POINT ( 'NONE',  ( -62.91457587699539289, 8.067188213978639055, 2.213507334852100055E-15 ) ) ;
#15612=CARTESIAN_POINT ( 'NONE',  ( -60.04781580374580585, 11.89276268270289982, -5.000000000000000000 ) ) ;
#15646=AXIS2_PLACEMENT_3D ( 'NONE', #4184, #11459, #15106 ) ;
#15682=VECTOR ( 'NONE', #3801, 1000.000000000000000 ) ;
#15704=DIRECTION ( 'NONE',  ( 0.005235963827117092427, -0.9999862922474493931, -2.636227439667000721E-16 ) ) ;
#15734=ORIENTED_EDGE ( 'NONE', *, *, #17029, .T. ) ;
#15813=LINE ( 'NONE', #2762, #12628 ) ;
#15820=CARTESIAN_POINT ( 'NONE',  ( -67.26895854462263458, 12.68829727884599201, 2.499999999999999556 ) ) ;
#15931=DIRECTION ( 'NONE',  ( 0.005235963827117092427, -0.9999862922474493931, -2.636227439667000721E-16 ) ) ;
#15964=SHAPE_REPRESENTATION ( 'Nut', ( #12739 ), #2264 ) ;
#15975=ORIENTED_EDGE ( 'NONE', *, *, #17769, .T. ) ;
#16030=CIRCLE ( 'NONE', #18714, 2.458500000000000352 ) ;
#16031=CYLINDRICAL_SURFACE ( 'NONE', #5818, 2.458500000000000352 ) ;
#16042=AXIS2_PLACEMENT_3D ( 'NONE', #15114, #7879, #11702 ) ;
#16066=CIRCLE ( 'NONE', #22828, 2.999765877365279998 ) ;
#16086=EDGE_CURVE ( 'NONE', #13198, #20578, #1258, .T. ) ;
#16168=CARTESIAN_POINT ( 'NONE',  ( -68.71210320717760567, 12.64039918458589895, 4.433884350144319916E-15 ) ) ;
#16203=VECTOR ( 'NONE', #17118, 1000.000000000000000 ) ;
#16240=( BOUNDED_CURVE ( )  B_SPLINE_CURVE ( 2, ( #3195, #5204, #8551 ),
 .UNSPECIFIED., .F., .F. ) 
 B_SPLINE_CURVE_WITH_KNOTS ( ( 3, 3 ),
 ( 0.000000000000000000, 0.5842180690389588982 ),
 .UNSPECIFIED. ) 
 CURVE ( )  GEOMETRIC_REPRESENTATION_ITEM ( )  RATIONAL_B_SPLINE_CURVE ( ( 1.000000000000000000, 1.154700538379249908, 1.000000000000000000 ) ) 
 REPRESENTATION_ITEM ( '' )  );
#16254=AXIS2_PLACEMENT_3D ( 'NONE', #9346, #14804, #17908 ) ;
#16321=DESIGN_CONTEXT ( 'detailed design', #924, 'design' ) ;
#16375=ADVANCED_FACE ( 'NONE', ( #23042 ), #6797, .F. ) ;
#16376=( BOUNDED_CURVE ( )  B_SPLINE_CURVE ( 2, ( #11714, #14776, #6237 ),
 .UNSPECIFIED., .F., .F. ) 
 B_SPLINE_CURVE_WITH_KNOTS ( ( 3, 3 ),
 ( 0.000000000000000000, 0.5842180690389578990 ),
 .UNSPECIFIED. ) 
 CURVE ( )  GEOMETRIC_REPRESENTATION_ITEM ( )  RATIONAL_B_SPLINE_CURVE ( ( 1.000000000000000000, 1.154700538379249908, 1.000000000000000000 ) ) 
 REPRESENTATION_ITEM ( '' )  );
#16428=ORIENTED_EDGE ( 'NONE', *, *, #16086, .T. ) ;
#16467=LINE ( 'NONE', #12912, #17319 ) ;
#16575=VECTOR ( 'NONE', #10131, 1000.000000000000000 ) ;
#16577=DIRECTION ( 'NONE',  ( -0.8686315144360597928, 0.4954586684361443893, 2.575384811085934765E-17 ) ) ;
#16607=LINE ( 'NONE', #2491, #18143 ) ;
#16626=EDGE_CURVE ( 'NONE', #14219, #6893, #20051, .T. ) ;
#16722=VERTEX_POINT ( 'NONE', #9274 ) ;
#16755=DIRECTION ( 'NONE',  ( 0.005235963827117092427, -0.9999862922474493931, -2.636227439667000721E-16 ) ) ;
#16772=ORIENTED_EDGE ( 'NONE', *, *, #16086, .F. ) ;
#16801=CARTESIAN_POINT ( 'NONE',  ( -68.02328523594360377, 12.24750435041217678, 3.945517663836197344E-15 ) ) ;
#16973=CARTESIAN_POINT ( 'NONE',  ( -58.60882321939761397, 12.73364205572179841, 2.500000000000008882 ) ) ;
#16996=CONICAL_SURFACE ( 'NONE', #23058, 5.086751345948125724, 1.047197551196598297 ) ;
#17029=EDGE_CURVE ( 'NONE', #22086, #11012, #2397, .T. ) ;
#17118=DIRECTION ( 'NONE',  ( 0.005235963827117092427, -0.9999862922474493931, -2.636227439667000721E-16 ) ) ;
#17203=DIRECTION ( 'NONE',  ( 0.8686315144360597928, -0.4954586684361442783, -1.318113719833499867E-16 ) ) ;
#17319=VECTOR ( 'NONE', #16577, 1000.000000000000114 ) ;
#17410=EDGE_CURVE ( 'NONE', #22086, #23172, #4771, .T. ) ;
#17495=DIRECTION ( 'NONE',  ( -0.005235963827117002221, 0.9999862922474493931, 2.636227439667000721E-16 ) ) ;
#17569=ORIENTED_EDGE ( 'NONE', *, *, #17410, .T. ) ;
#17616=CARTESIAN_POINT ( 'NONE',  ( -57.82789425897600211, 8.093822260023562976, 2.213507334852099266E-15 ) ) ;
#17632=DIRECTION ( 'NONE',  ( 1.000000000000000000, -1.380319151415139905E-18, 0.000000000000000000 ) ) ;
#17641=EDGE_LOOP ( 'NONE', ( #13339, #17569, #21356, #9536, #658, #22459 ) ) ;
#17714=ORIENTED_EDGE ( 'NONE', *, *, #9558, .T. ) ;
#17750=DIRECTION ( 'NONE',  ( 0.000000000000000000, 0.000000000000000000, -1.000000000000000000 ) ) ;
#17769=EDGE_CURVE ( 'NONE', #15538, #13655, #7375, .T. ) ;
#17778=( BOUNDED_CURVE ( )  B_SPLINE_CURVE ( 2, ( #21980, #3602, #21634 ),
 .UNSPECIFIED., .F., .F. ) 
 B_SPLINE_CURVE_WITH_KNOTS ( ( 3, 3 ),
 ( 0.000000000000000000, 0.5842180690389598974 ),
 .UNSPECIFIED. ) 
 CURVE ( )  GEOMETRIC_REPRESENTATION_ITEM ( )  RATIONAL_B_SPLINE_CURVE ( ( 1.000000000000000000, 1.154700538379249908, 1.000000000000000000 ) ) 
 REPRESENTATION_ITEM ( '' )  );
#17806=EDGE_CURVE ( 'NONE', #11097, #11763, #18411, .T. ) ;
#17869=ORIENTED_EDGE ( 'NONE', *, *, #2822, .F. ) ;
#17908=DIRECTION ( 'NONE',  ( 0.9999862922474493931, 0.005235963827117055998, -1.750845403988397166E-31 ) ) ;
#17928=VERTEX_POINT ( 'NONE', #12465 ) ;
#18036=ORIENTED_EDGE ( 'NONE', *, *, #10864, .F. ) ;
#18076=EDGE_CURVE ( 'NONE', #22844, #21777, #16066, .T. ) ;
#18143=VECTOR ( 'NONE', #4033, 1000.000000000000000 ) ;
#18153=ORIENTED_EDGE ( 'NONE', *, *, #4482, .T. ) ;
#18297=ORIENTED_EDGE ( 'NONE', *, *, #13271, .F. ) ;
#18411=( BOUNDED_CURVE ( )  B_SPLINE_CURVE ( 2, ( #19132, #16973, #2848 ),
 .UNSPECIFIED., .F., .F. ) 
 B_SPLINE_CURVE_WITH_KNOTS ( ( 3, 3 ),
 ( 0.000000000000000000, 0.5842180690389588982 ),
 .UNSPECIFIED. ) 
 CURVE ( )  GEOMETRIC_REPRESENTATION_ITEM ( )  RATIONAL_B_SPLINE_CURVE ( ( 1.000000000000000000, 1.154700538379249908, 1.000000000000000000 ) ) 
 REPRESENTATION_ITEM ( '' )  );
#18468=FACE_BOUND ( 'NONE', #11519, .T. ) ;
#18475=CARTESIAN_POINT ( 'NONE',  ( -68.69007546624879978, 8.433449002107520798, 2.873144230283079984E-15 ) ) ;
#18518=DIRECTION ( 'NONE',  ( 0.9999862922474491711, 0.005235963827117207786, -1.514467536079854800E-31 ) ) ;
#18543=EDGE_LOOP ( 'NONE', ( #3762, #20716, #10311, #9031 ) ) ;
#18636=ORIENTED_EDGE ( 'NONE', *, *, #5240, .F. ) ;
#18714=AXIS2_PLACEMENT_3D ( 'NONE', #22843, #13834, #17750 ) ;
#18715=CARTESIAN_POINT ( 'NONE',  ( -62.93867965702761325, 12.67062903583649991, 1.345427500395039956E-15 ) ) ;
#18748=VECTOR ( 'NONE', #12036, 1000.000000000000114 ) ;
#18790=ORIENTED_EDGE ( 'NONE', *, *, #4482, .F. ) ;
#18861=CARTESIAN_POINT ( 'NONE',  ( -62.93867965702758482, 12.67062903583649991, 2.999765877365342615 ) ) ;
#18864=ADVANCED_FACE ( 'NONE', ( #748 ), #8023, .T. ) ;
#18919=ORIENTED_EDGE ( 'NONE', *, *, #13921, .F. ) ;
#19019=EDGE_CURVE ( 'NONE', #11763, #14219, #23189, .T. ) ;
#19021=SHAPE_REPRESENTATION_RELATIONSHIP ( 'NONE' , 'NONE' ,  #15964, #2856 ) ;
#19132=CARTESIAN_POINT ( 'NONE',  ( -57.16110402867079898, 11.90787760832819941, 3.218044905330409686E-15 ) ) ;
#19143=DIRECTION ( 'NONE',  ( 0.005235963827117092427, -0.9999862922474493931, -2.636227439667000721E-16 ) ) ;
#19383=ORIENTED_EDGE ( 'NONE', *, *, #16626, .F. ) ;
#19385=CARTESIAN_POINT ( 'NONE',  ( -60.04781580374580585, 11.89276268270289982, 5.000000000000000000 ) ) ;
#19401=CARTESIAN_POINT ( 'NONE',  ( -60.02994014102380049, 8.478793778983318319, 5.000000000000000000 ) ) ;
#19441=( BOUNDED_CURVE ( )  B_SPLINE_CURVE ( 2, ( #4897, #15820, #22816 ),
 .UNSPECIFIED., .F., .F. ) 
 B_SPLINE_CURVE_WITH_KNOTS ( ( 3, 3 ),
 ( 0.000000000000000000, 0.5842180690389578990 ),
 .UNSPECIFIED. ) 
 CURVE ( )  GEOMETRIC_REPRESENTATION_ITEM ( )  RATIONAL_B_SPLINE_CURVE ( ( 1.000000000000000000, 1.154700538379249908, 1.000000000000000000 ) ) 
 REPRESENTATION_ITEM ( '' )  );
#19528=CARTESIAN_POINT ( 'NONE',  ( -60.05196788195259927, 12.68574396146170180, 5.000000000000000000 ) ) ;
#19783=DIRECTION ( 'NONE',  ( 0.000000000000000000, 0.000000000000000000, -1.000000000000000000 ) ) ;
#19784=ADVANCED_FACE ( 'NONE', ( #4131 ), #19805, .T. ) ;
#19802=ORIENTED_EDGE ( 'NONE', *, *, #21592, .T. ) ;
#19805=CONICAL_SURFACE ( 'NONE', #6159, 5.086751345948125724, 1.047197551196598297 ) ;
#19868=AXIS2_PLACEMENT_3D ( 'NONE', #8905, #21700, #1749 ) ;
#19913=AXIS2_PLACEMENT_3D ( 'NONE', #1873, #21852, #21962 ) ;
#19939=ORIENTED_EDGE ( 'NONE', *, *, #950, .F. ) ;
#19949=DIRECTION ( 'NONE',  ( 0.005235963827117092427, -0.9999862922474493931, -2.636227439667000721E-16 ) ) ;
#19963=EDGE_CURVE ( 'NONE', #11012, #11097, #11751, .T. ) ;
#20011=LINE ( 'NONE', #162, #202 ) ;
#20051=( BOUNDED_CURVE ( )  B_SPLINE_CURVE ( 2, ( #13188, #4152, #11423 ),
 .UNSPECIFIED., .F., .F. ) 
 B_SPLINE_CURVE_WITH_KNOTS ( ( 3, 3 ),
 ( 0.000000000000000000, 0.5842180690389588982 ),
 .UNSPECIFIED. ) 
 CURVE ( )  GEOMETRIC_REPRESENTATION_ITEM ( )  RATIONAL_B_SPLINE_CURVE ( ( 1.000000000000000000, 1.154700538379249908, 1.000000000000000000 ) ) 
 REPRESENTATION_ITEM ( '' )  );
#20078=LINE ( 'NONE', #16168, #15682 ) ;
#20126=CARTESIAN_POINT ( 'NONE',  ( -60.02994014102380049, 8.478793778983318319, 5.000000000000000000 ) ) ;
#20171=CARTESIAN_POINT ( 'NONE',  ( -62.93867965702761325, 12.67062903583649991, 3.427095671567209849E-15 ) ) ;
#20191=CARTESIAN_POINT ( 'NONE',  ( -65.80336369117380002, 8.448563927732790191, -5.000000000000000000 ) ) ;
#20282=CARTESIAN_POINT ( 'NONE',  ( -62.91249983789198552, 7.670697574599230073, 2.108981951733699973E-15 ) ) ;
#20578=VERTEX_POINT ( 'NONE', #15612 ) ;
#20716=ORIENTED_EDGE ( 'NONE', *, *, #7929, .F. ) ;
#20727=DIRECTION ( 'NONE',  ( 0.8660135325225010172, 0.004534477687579660174, 0.5000000000000000000 ) ) ;
#20730=AXIS2_PLACEMENT_3D ( 'NONE', #1334, #10405, #17632 ) ;
#20790=CARTESIAN_POINT ( 'NONE',  ( -65.80336369117380002, 8.448563927732790191, 5.000000000000000000 ) ) ;
#20826=ADVANCED_FACE ( 'NONE', ( #15353 ), #22103, .T. ) ;
#20873=CARTESIAN_POINT ( 'NONE',  ( -68.70795112897079093, 11.84741790582710053, 3.773156417642989929E-15 ) ) ;
#20908=ORIENTED_EDGE ( 'NONE', *, *, #118, .T. ) ;
#20941=VECTOR ( 'NONE', #607, 1000.000000000000114 ) ;
#20961=( BOUNDED_CURVE ( )  B_SPLINE_CURVE ( 2, ( #4520, #15335, #12027 ),
 .UNSPECIFIED., .F., .F. ) 
 B_SPLINE_CURVE_WITH_KNOTS ( ( 3, 3 ),
 ( 0.000000000000000000, 0.5842180690389578990 ),
 .UNSPECIFIED. ) 
 CURVE ( )  GEOMETRIC_REPRESENTATION_ITEM ( )  RATIONAL_B_SPLINE_CURVE ( ( 1.000000000000000000, 1.154700538379249908, 1.000000000000000000 ) ) 
 REPRESENTATION_ITEM ( '' )  );
#21020=ORIENTED_EDGE ( 'NONE', *, *, #11631, .T. ) ;
#21166=EDGE_CURVE ( 'NONE', #23172, #17928, #20078, .T. ) ;
#21234=ORIENTED_EDGE ( 'NONE', *, *, #10035, .F. ) ;
#21308=ORIENTED_EDGE ( 'NONE', *, *, #19019, .T. ) ;
#21356=ORIENTED_EDGE ( 'NONE', *, *, #6252, .F. ) ;
#21422=PRODUCT ( 'Nut', 'Nut', '', ( #1074 ) ) ;
#21496=EDGE_LOOP ( 'NONE', ( #16428, #1192, #2419, #585 ) ) ;
#21499=SHAPE_DEFINITION_REPRESENTATION ( #14017, #15964 ) ;
#21592=EDGE_CURVE ( 'NONE', #16722, #17928, #16467, .T. ) ;
#21601=CARTESIAN_POINT ( 'NONE',  ( -62.91331795724000386, 7.826945432762889787, 2.150173005478499992E-15 ) ) ;
#21634=CARTESIAN_POINT ( 'NONE',  ( -65.82123935389580538, 11.86253283145240012, -5.000000000000000000 ) ) ;
#21653=FACE_OUTER_BOUND ( 'NONE', #21496, .T. ) ;
#21700=DIRECTION ( 'NONE',  ( -0.005235963827117092427, 0.9999862922474493931, 2.636227439667000721E-16 ) ) ;
#21711=AXIS2_PLACEMENT_3D ( 'NONE', #3450, #8926, #12725 ) ;
#21721=CONICAL_SURFACE ( 'NONE', #14516, 2.729132938682640397, 1.047197551196598297 ) ;
#21733=DIRECTION ( 'NONE',  ( -0.005235963827117092427, 0.9999862922474493931, 2.636227439667000721E-16 ) ) ;
#21735=ORIENTED_EDGE ( 'NONE', *, *, #10864, .T. ) ;
#21777=VERTEX_POINT ( 'NONE', #18861 ) ;
#21852=DIRECTION ( 'NONE',  ( 0.8660135325225012393, 0.004534477687579934260, -0.4999999999999995004 ) ) ;
#21899=CARTESIAN_POINT ( 'NONE',  ( -65.80336369117380002, 8.448563927732790191, 5.000000000000000000 ) ) ;
#21908=AXIS2_PLACEMENT_3D ( 'NONE', #18715, #2301, #2181 ) ;
#21962=DIRECTION ( 'NONE',  ( 0.000000000000000000, -0.9999588795606764169, -0.009068582455730644573 ) ) ;
#21980=CARTESIAN_POINT ( 'NONE',  ( -68.70795112897079093, 11.84741790582710053, 3.773156417642989929E-15 ) ) ;
#21981=( BOUNDED_CURVE ( )  B_SPLINE_CURVE ( 2, ( #21899, #12881, #20126 ),
 .UNSPECIFIED., .F., .F. ) 
 B_SPLINE_CURVE_WITH_KNOTS ( ( 3, 3 ),
 ( 0.000000000000000000, 0.5842180690389598974 ),
 .UNSPECIFIED. ) 
 CURVE ( )  GEOMETRIC_REPRESENTATION_ITEM ( )  RATIONAL_B_SPLINE_CURVE ( ( 1.000000000000000000, 1.154700538379249908, 1.000000000000000000 ) ) 
 REPRESENTATION_ITEM ( '' )  );
#22018=VERTEX_POINT ( 'NONE', #4108 ) ;
#22086=VERTEX_POINT ( 'NONE', #2677 ) ;
#22103=CONICAL_SURFACE ( 'NONE', #16042, 5.086751345948125724, 1.047197551196598297 ) ;
#22220=FACE_OUTER_BOUND ( 'NONE', #8878, .T. ) ;
#22222=ADVANCED_FACE ( 'NONE', ( #759 ), #6250, .T. ) ;
#22291=PRODUCT_DEFINITION ( 'UNKNOWN', '', #7614, #16321 ) ;
#22336=ORIENTED_EDGE ( 'NONE', *, *, #10263, .T. ) ;
#22459=ORIENTED_EDGE ( 'NONE', *, *, #19963, .F. ) ;
#22570=CARTESIAN_POINT ( 'NONE',  ( -57.16110402867079898, 11.90787760832819941, 3.218044905330409686E-15 ) ) ;
#22596=DIRECTION ( 'NONE',  ( 0.005235963827117091560, -0.9999862922474493931, -2.636227439666999735E-16 ) ) ;
#22681=CARTESIAN_POINT ( 'NONE',  ( -65.82539143210260590, 12.65551411021120032, -5.000000000000000000 ) ) ;
#22711=DIRECTION ( 'NONE',  ( 0.9999862922474493931, 0.005235963827117055998, -1.750845403988397166E-31 ) ) ;
#22816=CARTESIAN_POINT ( 'NONE',  ( -68.70795112897079093, 11.84741790582710053, 3.773156417642989929E-15 ) ) ;
#22828=AXIS2_PLACEMENT_3D ( 'NONE', #20171, #7358, #1866 ) ;
#22839=CARTESIAN_POINT ( 'NONE',  ( -62.91249983789198552, 7.670697574599230073, 2.108981951733699973E-15 ) ) ;
#22843=CARTESIAN_POINT ( 'NONE',  ( -62.93704341833160498, 12.35813331950920002, 3.344713564077609812E-15 ) ) ;
#22844=VERTEX_POINT ( 'NONE', #14043 ) ;
#22899=AXIS2_PLACEMENT_3D ( 'NONE', #12329, #13732, #1004 ) ;
#23024=CIRCLE ( 'NONE', #8631, 4.399999999999997691 ) ;
#23042=FACE_OUTER_BOUND ( 'NONE', #18543, .T. ) ;
#23058=AXIS2_PLACEMENT_3D ( 'NONE', #15593, #17495, #15361 ) ;
#23162=LINE ( 'NONE', #1439, #4618 ) ;
#23172=VERTEX_POINT ( 'NONE', #20873 ) ;
#23189=LINE ( 'NONE', #19528, #12255 ) ;
#23323=DIRECTION ( 'NONE',  ( 2.306143273112860358E-15, 2.757014059715200372E-16, -1.000000000000000000 ) ) ;
#23377=DIRECTION ( 'NONE',  ( 0.005235963827117092427, -0.9999862922474493931, -2.636227439667000721E-16 ) ) ;
#23430=EDGE_LOOP ( 'NONE', ( #17869, #21234 ) ) ;
#23529=COLOUR_RGB('Sky Blue', 0.31764706, 0.68627451, 0.89019608);
#23530=FILL_AREA_STYLE_COLOUR('',#23529);
#23531=FILL_AREA_STYLE('',(#23530));
#23532=SURFACE_STYLE_FILL_AREA(#23531);
#23533=SURFACE_SIDE_STYLE('',(#23532));
#23534=SURFACE_STYLE_USAGE(.BOTH.,#23533);
#23535=PRESENTATION_STYLE_ASSIGNMENT((#23534));
#23565=STYLED_ITEM('',(#23535),#1933);
#23566=MECHANICAL_DESIGN_GEOMETRIC_PRESENTATION_REPRESENTATION('',(#23565),#2264);
ENDSEC;
END-ISO-10303-21;
